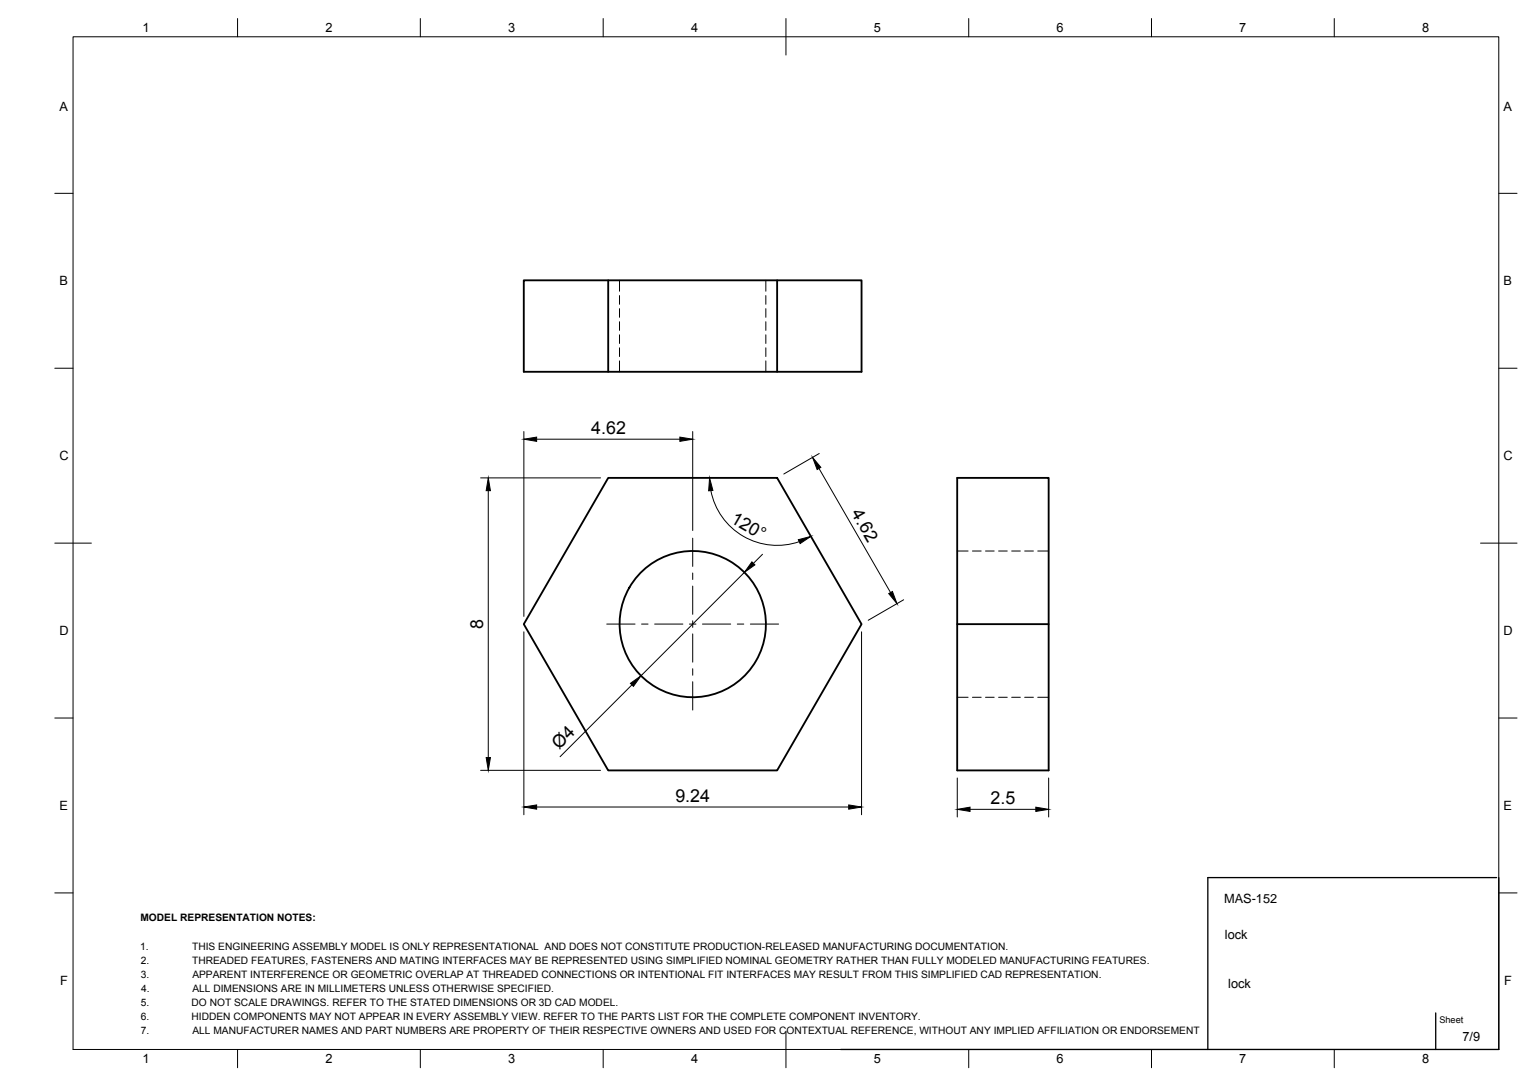
ISO-10303-21;
HEADER;
/* Generated by software containing ST-Developer
 * from STEP Tools, Inc. (www.steptools.com) 
 */

FILE_DESCRIPTION(
/* description */ ('STEP AP214'),
/* implementation_level */ '2;1');

FILE_NAME(
/* name */ 'lock.step',
/* time_stamp */ '2026-11-04T19:18:53-08:00',
/* author */ (''),
/* organization */ (''),
/* preprocessor_version */ 'ST-DEVELOPER v20.2',
/* originating_system */ 'Autodesk Translation Framework v15.17.0.0',
/* authorisation */ '');

FILE_SCHEMA (('AUTOMOTIVE_DESIGN { 1 0 10303 214 3 1 1 }'));
ENDSEC;

DATA;
#10=MECHANICAL_DESIGN_GEOMETRIC_PRESENTATION_REPRESENTATION('',(#84),#5942);
#70=SHAPE_REPRESENTATION_RELATIONSHIP('SRR','None',#5981,#77);
#77=ADVANCED_BREP_SHAPE_REPRESENTATION('',(#91),#5941);
#84=STYLED_ITEM('',(#6023),#91);
#91=MANIFOLD_SOLID_BREP('Body1',#931);
#98=FACE_BOUND('',#247,.T.);
#99=FACE_BOUND('',#249,.T.);
#132=PLANE('',#1092);
#133=PLANE('',#1093);
#134=PLANE('',#1094);
#135=PLANE('',#1095);
#136=PLANE('',#1096);
#137=PLANE('',#1097);
#138=PLANE('',#1098);
#139=PLANE('',#1099);
#185=FACE_OUTER_BOUND('',#245,.T.);
#186=FACE_OUTER_BOUND('',#246,.T.);
#187=FACE_OUTER_BOUND('',#248,.T.);
#188=FACE_OUTER_BOUND('',#250,.T.);
#189=FACE_OUTER_BOUND('',#251,.T.);
#190=FACE_OUTER_BOUND('',#252,.T.);
#191=FACE_OUTER_BOUND('',#253,.T.);
#192=FACE_OUTER_BOUND('',#254,.T.);
#193=FACE_OUTER_BOUND('',#255,.T.);
#245=EDGE_LOOP('',(#820,#821,#822,#823));
#246=EDGE_LOOP('',(#824,#825,#826,#827,#828,#829));
#247=EDGE_LOOP('',(#830));
#248=EDGE_LOOP('',(#831,#832,#833,#834,#835,#836));
#249=EDGE_LOOP('',(#837));
#250=EDGE_LOOP('',(#838,#839,#840,#841));
#251=EDGE_LOOP('',(#842,#843,#844,#845));
#252=EDGE_LOOP('',(#846,#847,#848,#849));
#253=EDGE_LOOP('',(#850,#851,#852,#853));
#254=EDGE_LOOP('',(#854,#855,#856,#857));
#255=EDGE_LOOP('',(#858,#859,#860,#861));
#315=LINE('',#5874,#393);
#316=LINE('',#5879,#394);
#317=LINE('',#5881,#395);
#318=LINE('',#5883,#396);
#319=LINE('',#5885,#397);
#320=LINE('',#5887,#398);
#321=LINE('',#5888,#399);
#322=LINE('',#5892,#400);
#323=LINE('',#5894,#401);
#324=LINE('',#5896,#402);
#325=LINE('',#5898,#403);
#326=LINE('',#5900,#404);
#327=LINE('',#5901,#405);
#328=LINE('',#5903,#406);
#329=LINE('',#5904,#407);
#330=LINE('',#5906,#408);
#331=LINE('',#5908,#409);
#332=LINE('',#5910,#410);
#333=LINE('',#5912,#411);
#393=VECTOR('',#1332,2.);
#394=VECTOR('',#1337,1000.);
#395=VECTOR('',#1338,1000.);
#396=VECTOR('',#1339,1000.);
#397=VECTOR('',#1340,1000.);
#398=VECTOR('',#1341,1000.);
#399=VECTOR('',#1342,1000.);
#400=VECTOR('',#1345,1000.);
#401=VECTOR('',#1346,1000.);
#402=VECTOR('',#1347,1000.);
#403=VECTOR('',#1348,1000.);
#404=VECTOR('',#1349,1000.);
#405=VECTOR('',#1350,1000.);
#406=VECTOR('',#1353,1000.);
#407=VECTOR('',#1354,1000.);
#408=VECTOR('',#1357,1000.);
#409=VECTOR('',#1360,1000.);
#410=VECTOR('',#1363,1000.);
#411=VECTOR('',#1366,1000.);
#442=CIRCLE('',#1090,2.);
#443=CIRCLE('',#1091,2.);
#506=VERTEX_POINT('',#5871);
#507=VERTEX_POINT('',#5873);
#508=VERTEX_POINT('',#5877);
#509=VERTEX_POINT('',#5878);
#510=VERTEX_POINT('',#5880);
#511=VERTEX_POINT('',#5882);
#512=VERTEX_POINT('',#5884);
#513=VERTEX_POINT('',#5886);
#514=VERTEX_POINT('',#5890);
#515=VERTEX_POINT('',#5891);
#516=VERTEX_POINT('',#5893);
#517=VERTEX_POINT('',#5895);
#518=VERTEX_POINT('',#5897);
#519=VERTEX_POINT('',#5899);
#613=EDGE_CURVE('',#506,#506,#442,.T.);
#614=EDGE_CURVE('',#506,#507,#315,.T.);
#615=EDGE_CURVE('',#507,#507,#443,.T.);
#616=EDGE_CURVE('',#508,#509,#316,.T.);
#617=EDGE_CURVE('',#509,#510,#317,.T.);
#618=EDGE_CURVE('',#510,#511,#318,.T.);
#619=EDGE_CURVE('',#511,#512,#319,.T.);
#620=EDGE_CURVE('',#512,#513,#320,.T.);
#621=EDGE_CURVE('',#513,#508,#321,.T.);
#622=EDGE_CURVE('',#514,#515,#322,.T.);
#623=EDGE_CURVE('',#516,#514,#323,.T.);
#624=EDGE_CURVE('',#517,#516,#324,.T.);
#625=EDGE_CURVE('',#518,#517,#325,.T.);
#626=EDGE_CURVE('',#519,#518,#326,.T.);
#627=EDGE_CURVE('',#515,#519,#327,.T.);
#628=EDGE_CURVE('',#509,#515,#328,.T.);
#629=EDGE_CURVE('',#508,#514,#329,.T.);
#630=EDGE_CURVE('',#510,#519,#330,.T.);
#631=EDGE_CURVE('',#511,#518,#331,.T.);
#632=EDGE_CURVE('',#512,#517,#332,.T.);
#633=EDGE_CURVE('',#513,#516,#333,.T.);
#820=ORIENTED_EDGE('',*,*,#613,.T.);
#821=ORIENTED_EDGE('',*,*,#614,.T.);
#822=ORIENTED_EDGE('',*,*,#615,.F.);
#823=ORIENTED_EDGE('',*,*,#614,.F.);
#824=ORIENTED_EDGE('',*,*,#616,.T.);
#825=ORIENTED_EDGE('',*,*,#617,.T.);
#826=ORIENTED_EDGE('',*,*,#618,.T.);
#827=ORIENTED_EDGE('',*,*,#619,.T.);
#828=ORIENTED_EDGE('',*,*,#620,.T.);
#829=ORIENTED_EDGE('',*,*,#621,.T.);
#830=ORIENTED_EDGE('',*,*,#613,.F.);
#831=ORIENTED_EDGE('',*,*,#622,.F.);
#832=ORIENTED_EDGE('',*,*,#623,.F.);
#833=ORIENTED_EDGE('',*,*,#624,.F.);
#834=ORIENTED_EDGE('',*,*,#625,.F.);
#835=ORIENTED_EDGE('',*,*,#626,.F.);
#836=ORIENTED_EDGE('',*,*,#627,.F.);
#837=ORIENTED_EDGE('',*,*,#615,.T.);
#838=ORIENTED_EDGE('',*,*,#622,.T.);
#839=ORIENTED_EDGE('',*,*,#628,.F.);
#840=ORIENTED_EDGE('',*,*,#616,.F.);
#841=ORIENTED_EDGE('',*,*,#629,.T.);
#842=ORIENTED_EDGE('',*,*,#627,.T.);
#843=ORIENTED_EDGE('',*,*,#630,.F.);
#844=ORIENTED_EDGE('',*,*,#617,.F.);
#845=ORIENTED_EDGE('',*,*,#628,.T.);
#846=ORIENTED_EDGE('',*,*,#626,.T.);
#847=ORIENTED_EDGE('',*,*,#631,.F.);
#848=ORIENTED_EDGE('',*,*,#618,.F.);
#849=ORIENTED_EDGE('',*,*,#630,.T.);
#850=ORIENTED_EDGE('',*,*,#625,.T.);
#851=ORIENTED_EDGE('',*,*,#632,.F.);
#852=ORIENTED_EDGE('',*,*,#619,.F.);
#853=ORIENTED_EDGE('',*,*,#631,.T.);
#854=ORIENTED_EDGE('',*,*,#624,.T.);
#855=ORIENTED_EDGE('',*,*,#633,.F.);
#856=ORIENTED_EDGE('',*,*,#620,.F.);
#857=ORIENTED_EDGE('',*,*,#632,.T.);
#858=ORIENTED_EDGE('',*,*,#623,.T.);
#859=ORIENTED_EDGE('',*,*,#629,.F.);
#860=ORIENTED_EDGE('',*,*,#621,.F.);
#861=ORIENTED_EDGE('',*,*,#633,.T.);
#870=CYLINDRICAL_SURFACE('',#1089,2.);
#916=ADVANCED_FACE('',(#185),#870,.F.);
#917=ADVANCED_FACE('',(#186,#98),#132,.T.);
#918=ADVANCED_FACE('',(#187,#99),#133,.F.);
#919=ADVANCED_FACE('',(#188),#134,.F.);
#920=ADVANCED_FACE('',(#189),#135,.F.);
#921=ADVANCED_FACE('',(#190),#136,.F.);
#922=ADVANCED_FACE('',(#191),#137,.F.);
#923=ADVANCED_FACE('',(#192),#138,.F.);
#924=ADVANCED_FACE('',(#193),#139,.F.);
#931=CLOSED_SHELL('',(#916,#917,#918,#919,#920,#921,#922,#923,#924));
#1088=AXIS2_PLACEMENT_3D('',#5869,#1326,#1327);
#1089=AXIS2_PLACEMENT_3D('',#5870,#1328,#1329);
#1090=AXIS2_PLACEMENT_3D('',#5872,#1330,#1331);
#1091=AXIS2_PLACEMENT_3D('',#5875,#1333,#1334);
#1092=AXIS2_PLACEMENT_3D('',#5876,#1335,#1336);
#1093=AXIS2_PLACEMENT_3D('',#5889,#1343,#1344);
#1094=AXIS2_PLACEMENT_3D('',#5902,#1351,#1352);
#1095=AXIS2_PLACEMENT_3D('',#5905,#1355,#1356);
#1096=AXIS2_PLACEMENT_3D('',#5907,#1358,#1359);
#1097=AXIS2_PLACEMENT_3D('',#5909,#1361,#1362);
#1098=AXIS2_PLACEMENT_3D('',#5911,#1364,#1365);
#1099=AXIS2_PLACEMENT_3D('',#5913,#1367,#1368);
#1326=DIRECTION('axis',(0.,0.,1.));
#1327=DIRECTION('refdir',(1.,0.,0.));
#1328=DIRECTION('center_axis',(0.,0.,-1.));
#1329=DIRECTION('ref_axis',(-1.,0.,0.));
#1330=DIRECTION('center_axis',(0.,0.,1.));
#1331=DIRECTION('ref_axis',(1.,0.,0.));
#1332=DIRECTION('',(0.,0.,-1.));
#1333=DIRECTION('center_axis',(0.,0.,1.));
#1334=DIRECTION('ref_axis',(1.,0.,0.));
#1335=DIRECTION('center_axis',(0.,0.,1.));
#1336=DIRECTION('ref_axis',(1.,0.,0.));
#1337=DIRECTION('',(0.,1.,0.));
#1338=DIRECTION('',(-0.866025403784439,0.5,0.));
#1339=DIRECTION('',(-0.866025403784438,-0.5,0.));
#1340=DIRECTION('',(0.,-1.,0.));
#1341=DIRECTION('',(0.866025403784438,-0.5,0.));
#1342=DIRECTION('',(0.866025403784438,0.5,0.));
#1343=DIRECTION('center_axis',(0.,0.,1.));
#1344=DIRECTION('ref_axis',(1.,0.,0.));
#1345=DIRECTION('',(0.,1.,0.));
#1346=DIRECTION('',(0.866025403784438,0.5,0.));
#1347=DIRECTION('',(0.866025403784438,-0.5,0.));
#1348=DIRECTION('',(0.,-1.,0.));
#1349=DIRECTION('',(-0.866025403784438,-0.5,0.));
#1350=DIRECTION('',(-0.866025403784439,0.5,0.));
#1351=DIRECTION('center_axis',(-1.,0.,0.));
#1352=DIRECTION('ref_axis',(0.,0.,1.));
#1353=DIRECTION('',(0.,0.,-1.));
#1354=DIRECTION('',(0.,0.,-1.));
#1355=DIRECTION('center_axis',(-0.5,-0.866025403784439,0.));
#1356=DIRECTION('ref_axis',(0.866025403784439,-0.5,0.));
#1357=DIRECTION('',(0.,0.,-1.));
#1358=DIRECTION('center_axis',(0.5,-0.866025403784439,0.));
#1359=DIRECTION('ref_axis',(0.866025403784439,0.5,0.));
#1360=DIRECTION('',(0.,0.,-1.));
#1361=DIRECTION('center_axis',(1.,0.,0.));
#1362=DIRECTION('ref_axis',(0.,0.,-1.));
#1363=DIRECTION('',(0.,0.,-1.));
#1364=DIRECTION('center_axis',(0.5,0.866025403784439,0.));
#1365=DIRECTION('ref_axis',(-0.866025403784439,0.5,0.));
#1366=DIRECTION('',(0.,0.,-1.));
#1367=DIRECTION('center_axis',(-0.5,0.866025403784438,0.));
#1368=DIRECTION('ref_axis',(-0.866025403784438,-0.5,0.));
#5869=CARTESIAN_POINT('',(0.,0.,0.));
#5870=CARTESIAN_POINT('Origin',(0.,0.,4.5));
#5871=CARTESIAN_POINT('',(2.,-2.44929359829471E-16,4.5));
#5872=CARTESIAN_POINT('Origin',(0.,0.,4.5));
#5873=CARTESIAN_POINT('',(2.,-2.44929359829471E-16,2.));
#5874=CARTESIAN_POINT('',(2.,-2.44929359829471E-16,4.5));
#5875=CARTESIAN_POINT('Origin',(0.,0.,2.));
#5876=CARTESIAN_POINT('Origin',(0.,0.,4.5));
#5877=CARTESIAN_POINT('',(4.,-2.3094010767585,4.5));
#5878=CARTESIAN_POINT('',(4.,2.3094010767585,4.5));
#5879=CARTESIAN_POINT('',(4.,-2.3094010767585,4.5));
#5880=CARTESIAN_POINT('',(-1.32814766129474E-15,4.61880215351701,4.5));
#5881=CARTESIAN_POINT('',(4.,2.3094010767585,4.5));
#5882=CARTESIAN_POINT('',(-4.,2.3094010767585,4.5));
#5883=CARTESIAN_POINT('',(-1.32814766129474E-15,4.61880215351701,4.5));
#5884=CARTESIAN_POINT('',(-4.,-2.3094010767585,4.5));
#5885=CARTESIAN_POINT('',(-4.,2.3094010767585,4.5));
#5886=CARTESIAN_POINT('',(3.45589442479754E-15,-4.61880215351701,4.5));
#5887=CARTESIAN_POINT('',(-4.,-2.3094010767585,4.5));
#5888=CARTESIAN_POINT('',(3.45589442479754E-15,-4.61880215351701,4.5));
#5889=CARTESIAN_POINT('Origin',(0.,0.,2.));
#5890=CARTESIAN_POINT('',(4.,-2.3094010767585,2.));
#5891=CARTESIAN_POINT('',(4.,2.3094010767585,2.));
#5892=CARTESIAN_POINT('',(4.,-2.3094010767585,2.));
#5893=CARTESIAN_POINT('',(3.45589442479754E-15,-4.61880215351701,2.));
#5894=CARTESIAN_POINT('',(3.45589442479754E-15,-4.61880215351701,2.));
#5895=CARTESIAN_POINT('',(-4.,-2.3094010767585,2.));
#5896=CARTESIAN_POINT('',(-4.,-2.3094010767585,2.));
#5897=CARTESIAN_POINT('',(-4.,2.3094010767585,2.));
#5898=CARTESIAN_POINT('',(-4.,2.3094010767585,2.));
#5899=CARTESIAN_POINT('',(-1.32814766129474E-15,4.61880215351701,2.));
#5900=CARTESIAN_POINT('',(-1.32814766129474E-15,4.61880215351701,2.));
#5901=CARTESIAN_POINT('',(4.,2.3094010767585,2.));
#5902=CARTESIAN_POINT('Origin',(4.,-2.3094010767585,4.5));
#5903=CARTESIAN_POINT('',(4.,2.3094010767585,4.5));
#5904=CARTESIAN_POINT('',(4.,-2.3094010767585,4.5));
#5905=CARTESIAN_POINT('Origin',(4.,2.3094010767585,4.5));
#5906=CARTESIAN_POINT('',(-1.32814766129474E-15,4.61880215351701,4.5));
#5907=CARTESIAN_POINT('Origin',(-1.32814766129474E-15,4.61880215351701,
4.5));
#5908=CARTESIAN_POINT('',(-4.,2.3094010767585,4.5));
#5909=CARTESIAN_POINT('Origin',(-4.,2.3094010767585,4.5));
#5910=CARTESIAN_POINT('',(-4.,-2.3094010767585,4.5));
#5911=CARTESIAN_POINT('Origin',(-4.,-2.3094010767585,4.5));
#5912=CARTESIAN_POINT('',(3.45589442479754E-15,-4.61880215351701,4.5));
#5913=CARTESIAN_POINT('Origin',(3.45589442479754E-15,-4.61880215351701,
4.5));
#5932=UNCERTAINTY_MEASURE_WITH_UNIT(LENGTH_MEASURE(0.01),#5943,
'DISTANCE_ACCURACY_VALUE',
'Maximum model space distance between geometric entities at asserted c
onnectivities');
#5933=UNCERTAINTY_MEASURE_WITH_UNIT(LENGTH_MEASURE(0.01),#5943,
'DISTANCE_ACCURACY_VALUE',
'Maximum model space distance between geometric entities at asserted c
onnectivities');
#5941=(
GEOMETRIC_REPRESENTATION_CONTEXT(3)
GLOBAL_UNCERTAINTY_ASSIGNED_CONTEXT((#5932))
GLOBAL_UNIT_ASSIGNED_CONTEXT((#5943,#5945,#5946))
REPRESENTATION_CONTEXT('','3D')
);
#5942=(
GEOMETRIC_REPRESENTATION_CONTEXT(3)
GLOBAL_UNCERTAINTY_ASSIGNED_CONTEXT((#5933))
GLOBAL_UNIT_ASSIGNED_CONTEXT((#5943,#5945,#5946))
REPRESENTATION_CONTEXT('','3D')
);
#5943=(
LENGTH_UNIT()
NAMED_UNIT(*)
SI_UNIT(.MILLI.,.METRE.)
);
#5945=(
NAMED_UNIT(*)
PLANE_ANGLE_UNIT()
SI_UNIT($,.RADIAN.)
);
#5946=(
NAMED_UNIT(*)
SI_UNIT($,.STERADIAN.)
SOLID_ANGLE_UNIT()
);
#5954=SHAPE_DEFINITION_REPRESENTATION(#5962,#5981);
#5962=PRODUCT_DEFINITION_SHAPE('',$,#5990);
#5981=SHAPE_REPRESENTATION('',(#1088),#5941);
#5982=PRODUCT_DEFINITION_CONTEXT('part definition',#6008,'design');
#5990=PRODUCT_DEFINITION('lock','lock',#5998,#5982);
#5998=PRODUCT_DEFINITION_FORMATION('',$,#6017);
#6008=APPLICATION_CONTEXT(
'Core Data for Automotive Mechanical Design Process');
#6009=PRODUCT_CONTEXT('part definition',#6008,'mechanical');
#6017=PRODUCT('lock','lock',$,(#6009));
#6023=PRESENTATION_STYLE_ASSIGNMENT((#6029));
#6029=SURFACE_STYLE_USAGE(.BOTH.,#6035);
#6035=SURFACE_SIDE_STYLE('',(#6041));
#6041=SURFACE_STYLE_FILL_AREA(#6047);
#6047=FILL_AREA_STYLE('Opaque(61,176,222)',(#6053));
#6053=FILL_AREA_STYLE_COLOUR('Opaque(61,176,222)',#6059);
#6059=COLOUR_RGB('Opaque(61,176,222)',0.23921568627451,0.690196078431373,
0.870588235294118);
ENDSEC;
END-ISO-10303-21;
